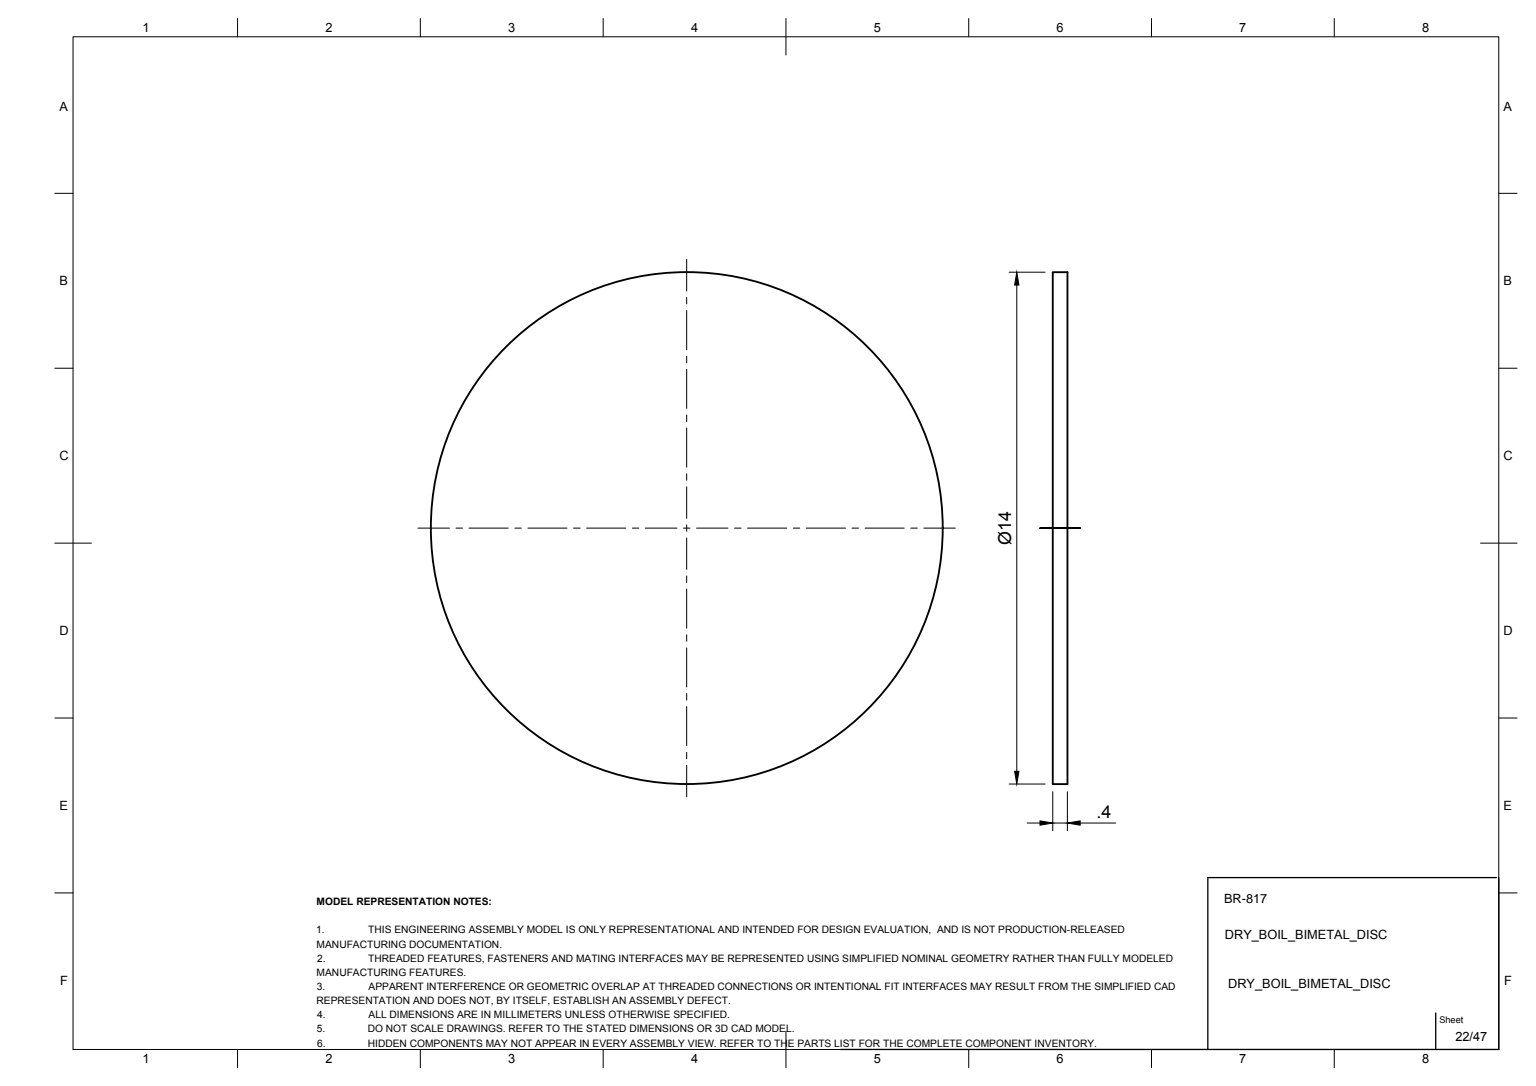
ISO-10303-21;
HEADER;
FILE_DESCRIPTION((''),'2;1');
FILE_NAME('DRY_BOIL_BIMETAL_DISC.step','2026-10-01T22:07:29-07:00',(''),(''),'','','');
FILE_SCHEMA (('AUTOMOTIVE_DESIGN { 1 0 10303 214 3 1 1 }'));
ENDSEC;
DATA;
#10=MECHANICAL_DESIGN_GEOMETRIC_PRESENTATION_REPRESENTATION('',(#556),#15484);
#486=SHAPE_REPRESENTATION_RELATIONSHIP('SRR','None',#15635,#521) ;
#521=ADVANCED_BREP_SHAPE_REPRESENTATION('',(#597),#15459) ;
#556=STYLED_ITEM('',(#15835),#597) ;
#597=MANIFOLD_SOLID_BREP('DRY_BOIL_BIMETAL_DISC',#8267) ;
#680=CYLINDRICAL_SURFACE('',#8990,0.7) ;
#1003=CIRCLE('',#8991,0.7) ;
#1004=CIRCLE('',#8992,0.7) ;
#1529=FACE_OUTER_BOUND('',#2085,.T.) ;
#1530=FACE_OUTER_BOUND('',#2086,.T.) ;
#1531=FACE_OUTER_BOUND('',#2087,.T.) ;
#2085=EDGE_LOOP('',(#5931,#5932,#5933,#5934)) ;
#2086=EDGE_LOOP('',(#5935)) ;
#2087=EDGE_LOOP('',(#5936)) ;
#2647=LINE('',#13669,#3121) ;
#3121=VECTOR('',#10752,0.7) ;
#3609=VERTEX_POINT('',#13666) ;
#3610=VERTEX_POINT('',#13668) ;
#4470=EDGE_CURVE('',#3609,#3609,#1003,.T.) ;
#4471=EDGE_CURVE('',#3609,#3610,#2647,.T.) ;
#4472=EDGE_CURVE('',#3610,#3610,#1004,.T.) ;
#5931=ORIENTED_EDGE('',*,*,#4470,.F.) ;
#5932=ORIENTED_EDGE('',*,*,#4471,.T.) ;
#5933=ORIENTED_EDGE('',*,*,#4472,.F.) ;
#5934=ORIENTED_EDGE('',*,*,#4471,.F.) ;
#5935=ORIENTED_EDGE('',*,*,#4472,.T.) ;
#5936=ORIENTED_EDGE('',*,*,#4470,.T.) ;
#7641=PLANE('',#8993) ;
#7642=PLANE('',#8994) ;
#7916=ADVANCED_FACE('',(#1529),#680,.T.) ;
#7917=ADVANCED_FACE('',(#1530),#7641,.T.) ;
#7918=ADVANCED_FACE('',(#1531),#7642,.T.) ;
#8267=CLOSED_SHELL('',(#7916,#7917,#7918)) ;
#8989=AXIS2_PLACEMENT_3D('',#13664,#10746,#10747) ;
#8990=AXIS2_PLACEMENT_3D('',#13665,#10748,#10749) ;
#8991=AXIS2_PLACEMENT_3D('',#13667,#10750,#10751) ;
#8992=AXIS2_PLACEMENT_3D('',#13670,#10753,#10754) ;
#8993=AXIS2_PLACEMENT_3D('',#13671,#10755,#10756) ;
#8994=AXIS2_PLACEMENT_3D('',#13672,#10757,#10758) ;
#10746=DIRECTION('axis',(0.,0.,1.)) ;
#10747=DIRECTION('refdir',(1.,0.,0.)) ;
#10748=DIRECTION('center_axis',(0.,0.,1.)) ;
#10749=DIRECTION('ref_axis',(1.,0.,0.)) ;
#10750=DIRECTION('center_axis',(0.,0.,1.)) ;
#10751=DIRECTION('ref_axis',(1.,0.,0.)) ;
#10752=DIRECTION('',(0.,0.,-1.)) ;
#10753=DIRECTION('center_axis',(0.,0.,-1.)) ;
#10754=DIRECTION('ref_axis',(1.,0.,0.)) ;
#10755=DIRECTION('center_axis',(0.,0.,-1.)) ;
#10756=DIRECTION('ref_axis',(-1.,0.,0.)) ;
#10757=DIRECTION('center_axis',(0.,0.,1.)) ;
#10758=DIRECTION('ref_axis',(1.,0.,0.)) ;
#13664=CARTESIAN_POINT('',(0.,0.,0.)) ;
#13665=CARTESIAN_POINT('Origin',(0.,-1.4,1.27)) ;
#13666=CARTESIAN_POINT('',(-0.7,-1.4,1.29)) ;
#13667=CARTESIAN_POINT('Origin',(0.,-1.4,1.29)) ;
#13668=CARTESIAN_POINT('',(-0.7,-1.4,1.25)) ;
#13669=CARTESIAN_POINT('',(-0.7,-1.4,1.27)) ;
#13670=CARTESIAN_POINT('Origin',(0.,-1.4,1.25)) ;
#13671=CARTESIAN_POINT('Origin',(0.,-1.4,1.25)) ;
#13672=CARTESIAN_POINT('Origin',(0.,-1.4,1.29)) ;
#15416=UNCERTAINTY_MEASURE_WITH_UNIT(LENGTH_MEASURE(0.001),#15485,
'DISTANCE_ACCURACY_VALUE',
'Maximum model space distance between geometric entities at asserted c
onnectivities') ;
#15441=UNCERTAINTY_MEASURE_WITH_UNIT(LENGTH_MEASURE(0.001),#15485,
'DISTANCE_ACCURACY_VALUE',
'Maximum model space distance between geometric entities at asserted c
onnectivities') ;
#15459=(
GEOMETRIC_REPRESENTATION_CONTEXT(3)
GLOBAL_UNCERTAINTY_ASSIGNED_CONTEXT((#15416))
GLOBAL_UNIT_ASSIGNED_CONTEXT((#15485,#15487,#15488))
REPRESENTATION_CONTEXT('','3D')
) ;
#15484=(
GEOMETRIC_REPRESENTATION_CONTEXT(3)
GLOBAL_UNCERTAINTY_ASSIGNED_CONTEXT((#15441))
GLOBAL_UNIT_ASSIGNED_CONTEXT((#15485,#15487,#15488))
REPRESENTATION_CONTEXT('','3D')
) ;
#15485=(
LENGTH_UNIT()
NAMED_UNIT(*)
SI_UNIT(.CENTI.,.METRE.)
) ;
#15487=(
NAMED_UNIT(*)
PLANE_ANGLE_UNIT()
SI_UNIT($,.RADIAN.)
) ;
#15488=(
NAMED_UNIT(*)
SI_UNIT($,.STERADIAN.)
SOLID_ANGLE_UNIT()
) ;
#15506=SHAPE_DEFINITION_REPRESENTATION(#15554,#15635) ;
#15554=PRODUCT_DEFINITION_SHAPE('',$,#15678) ;
#15635=SHAPE_REPRESENTATION('',(#8989),#15459) ;
#15660=PRODUCT_DEFINITION_CONTEXT('part definition',#15788,'design') ;
#15678=PRODUCT_DEFINITION('DRY_BOIL_BIMETAL_DISC',
'DRY_BOIL_BIMETAL_DISC',#15720,#15660) ;
#15720=PRODUCT_DEFINITION_FORMATION('',$,#15807) ;
#15788=APPLICATION_CONTEXT(
'Core Data for Automotive Mechanical Design Process') ;
#15789=PRODUCT_CONTEXT('part definition',#15788,'mechanical') ;
#15807=PRODUCT('DRY_BOIL_BIMETAL_DISC','DRY_BOIL_BIMETAL_DISC',$,(#15789)) ;
#15835=PRESENTATION_STYLE_ASSIGNMENT((#15847)) ;
#15847=SURFACE_STYLE_USAGE(.BOTH.,#15859) ;
#15859=SURFACE_SIDE_STYLE('',(#15871)) ;
#15871=SURFACE_STYLE_FILL_AREA(#15883) ;
#15883=FILL_AREA_STYLE('Stainless Steel - Satin',(#15895)) ;
#15895=FILL_AREA_STYLE_COLOUR('Stainless Steel - Satin',#15907) ;
#15907=COLOUR_RGB('Stainless Steel - Satin', 0.40784314, 0.44705882, 0.49803922) ;
ENDSEC;
END-ISO-10303-21;
